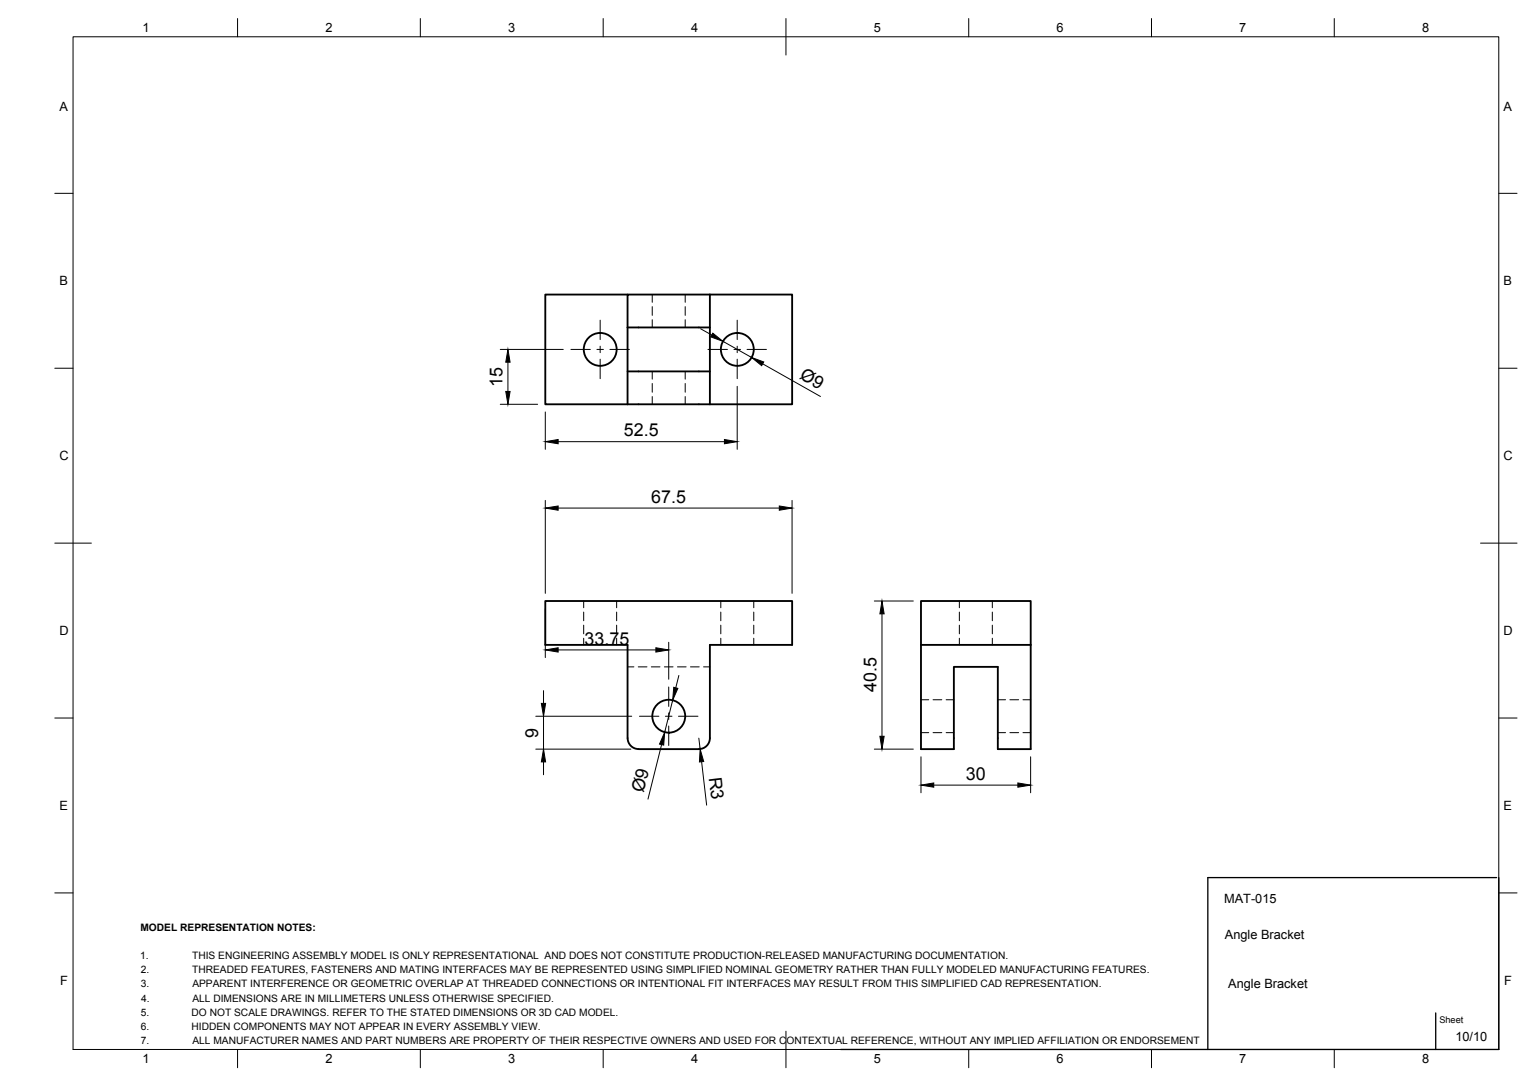
ISO-10303-21;
HEADER;
/* Generated by software containing ST-Developer
 * from STEP Tools, Inc. (www.steptools.com) 
 */

FILE_DESCRIPTION(
/* description */ ('STEP AP214'),
/* implementation_level */ '2;1');

FILE_NAME(
/* name */ 'Angle Bracket.step',
/* time_stamp */ '2026-11-14T06:03:18-08:00',
/* author */ (''),
/* organization */ (''),
/* preprocessor_version */ 'ST-DEVELOPER v20.2',
/* originating_system */ 'Autodesk Translation Framework v15.17.0.0',
/* authorisation */ '');

FILE_SCHEMA (('AUTOMOTIVE_DESIGN { 1 0 10303 214 3 1 1 }'));
ENDSEC;

DATA;
#10=MECHANICAL_DESIGN_GEOMETRIC_PRESENTATION_REPRESENTATION('',(#78),#3206);
#62=SHAPE_REPRESENTATION_RELATIONSHIP('SRR','None',#3245,#70);
#70=ADVANCED_BREP_SHAPE_REPRESENTATION('',(#86),#3204);
#78=STYLED_ITEM('',(#3290),#86);
#86=MANIFOLD_SOLID_BREP('Body1',#1785);
#131=PLANE('',#2029);
#132=PLANE('',#2030);
#133=PLANE('',#2031);
#134=PLANE('',#2032);
#135=PLANE('',#2033);
#136=PLANE('',#2034);
#137=PLANE('',#2037);
#138=PLANE('',#2038);
#139=PLANE('',#2041);
#140=PLANE('',#2042);
#141=PLANE('',#2043);
#142=PLANE('',#2044);
#143=PLANE('',#2047);
#144=PLANE('',#2050);
#180=FACE_BOUND('',#724,.T.);
#181=FACE_BOUND('',#726,.T.);
#182=FACE_BOUND('',#728,.T.);
#183=FACE_BOUND('',#729,.T.);
#184=FACE_BOUND('',#732,.T.);
#185=FACE_BOUND('',#735,.T.);
#186=FACE_BOUND('',#740,.T.);
#187=FACE_BOUND('',#742,.T.);
#286=LINE('',#3041,#431);
#287=LINE('',#3047,#432);
#288=LINE('',#3053,#433);
#289=LINE('',#3059,#434);
#290=LINE('',#3064,#435);
#291=LINE('',#3066,#436);
#292=LINE('',#3068,#437);
#293=LINE('',#3069,#438);
#294=LINE('',#3073,#439);
#295=LINE('',#3075,#440);
#296=LINE('',#3077,#441);
#297=LINE('',#3078,#442);
#298=LINE('',#3082,#443);
#299=LINE('',#3084,#444);
#300=LINE('',#3086,#445);
#301=LINE('',#3087,#446);
#302=LINE('',#3091,#447);
#303=LINE('',#3093,#448);
#304=LINE('',#3095,#449);
#305=LINE('',#3096,#450);
#306=LINE('',#3098,#451);
#307=LINE('',#3099,#452);
#308=LINE('',#3102,#453);
#309=LINE('',#3106,#454);
#310=LINE('',#3107,#455);
#311=LINE('',#3109,#456);
#312=LINE('',#3113,#457);
#313=LINE('',#3116,#458);
#314=LINE('',#3118,#459);
#315=LINE('',#3123,#460);
#316=LINE('',#3124,#461);
#317=LINE('',#3126,#462);
#318=LINE('',#3128,#463);
#319=LINE('',#3129,#464);
#320=LINE('',#3132,#465);
#321=LINE('',#3134,#466);
#322=LINE('',#3136,#467);
#323=LINE('',#3138,#468);
#324=LINE('',#3139,#469);
#325=LINE('',#3143,#470);
#326=LINE('',#3144,#471);
#327=LINE('',#3145,#472);
#328=LINE('',#3148,#473);
#329=LINE('',#3153,#474);
#431=VECTOR('',#2459,4.50000000000001);
#432=VECTOR('',#2466,4.50000000000001);
#433=VECTOR('',#2473,4.50000000000002);
#434=VECTOR('',#2480,4.50000000000001);
#435=VECTOR('',#2485,1000.);
#436=VECTOR('',#2486,1000.);
#437=VECTOR('',#2487,1000.);
#438=VECTOR('',#2488,1000.);
#439=VECTOR('',#2491,1000.);
#440=VECTOR('',#2492,1000.);
#441=VECTOR('',#2493,1000.);
#442=VECTOR('',#2494,1000.);
#443=VECTOR('',#2497,1000.);
#444=VECTOR('',#2498,1000.);
#445=VECTOR('',#2499,1000.);
#446=VECTOR('',#2500,1000.);
#447=VECTOR('',#2503,1000.);
#448=VECTOR('',#2504,1000.);
#449=VECTOR('',#2505,1000.);
#450=VECTOR('',#2506,1000.);
#451=VECTOR('',#2509,1000.);
#452=VECTOR('',#2510,1000.);
#453=VECTOR('',#2513,1000.);
#454=VECTOR('',#2518,1000.);
#455=VECTOR('',#2519,1000.);
#456=VECTOR('',#2522,1000.);
#457=VECTOR('',#2525,1000.);
#458=VECTOR('',#2528,1000.);
#459=VECTOR('',#2529,1000.);
#460=VECTOR('',#2534,1000.);
#461=VECTOR('',#2535,1000.);
#462=VECTOR('',#2536,1000.);
#463=VECTOR('',#2537,1000.);
#464=VECTOR('',#2538,1000.);
#465=VECTOR('',#2541,1000.);
#466=VECTOR('',#2542,1000.);
#467=VECTOR('',#2543,1000.);
#468=VECTOR('',#2544,1000.);
#469=VECTOR('',#2545,1000.);
#470=VECTOR('',#2548,1000.);
#471=VECTOR('',#2549,1000.);
#472=VECTOR('',#2550,1000.);
#473=VECTOR('',#2555,1000.);
#474=VECTOR('',#2564,1000.);
#503=CYLINDRICAL_SURFACE('',#2017,4.50000000000001);
#504=CYLINDRICAL_SURFACE('',#2020,4.50000000000001);
#505=CYLINDRICAL_SURFACE('',#2023,4.50000000000002);
#506=CYLINDRICAL_SURFACE('',#2026,4.50000000000001);
#507=CYLINDRICAL_SURFACE('',#2051,3.00000000000001);
#508=CYLINDRICAL_SURFACE('',#2052,3.00000000000001);
#509=CYLINDRICAL_SURFACE('',#2053,3.00000000000001);
#510=CYLINDRICAL_SURFACE('',#2054,3.00000000000001);
#585=FACE_OUTER_BOUND('',#718,.T.);
#586=FACE_OUTER_BOUND('',#719,.T.);
#587=FACE_OUTER_BOUND('',#720,.T.);
#588=FACE_OUTER_BOUND('',#721,.T.);
#589=FACE_OUTER_BOUND('',#722,.T.);
#590=FACE_OUTER_BOUND('',#723,.T.);
#591=FACE_OUTER_BOUND('',#725,.T.);
#592=FACE_OUTER_BOUND('',#727,.T.);
#593=FACE_OUTER_BOUND('',#730,.T.);
#594=FACE_OUTER_BOUND('',#731,.T.);
#595=FACE_OUTER_BOUND('',#733,.T.);
#596=FACE_OUTER_BOUND('',#734,.T.);
#597=FACE_OUTER_BOUND('',#736,.T.);
#598=FACE_OUTER_BOUND('',#737,.T.);
#599=FACE_OUTER_BOUND('',#738,.T.);
#600=FACE_OUTER_BOUND('',#739,.T.);
#601=FACE_OUTER_BOUND('',#741,.T.);
#602=FACE_OUTER_BOUND('',#743,.T.);
#603=FACE_OUTER_BOUND('',#744,.T.);
#604=FACE_OUTER_BOUND('',#745,.T.);
#605=FACE_OUTER_BOUND('',#746,.T.);
#606=FACE_OUTER_BOUND('',#747,.T.);
#718=EDGE_LOOP('',(#1541,#1542,#1543,#1544));
#719=EDGE_LOOP('',(#1545,#1546,#1547,#1548));
#720=EDGE_LOOP('',(#1549,#1550,#1551,#1552));
#721=EDGE_LOOP('',(#1553,#1554,#1555,#1556));
#722=EDGE_LOOP('',(#1557,#1558,#1559,#1560));
#723=EDGE_LOOP('',(#1561,#1562,#1563,#1564));
#724=EDGE_LOOP('',(#1565));
#725=EDGE_LOOP('',(#1566,#1567,#1568,#1569));
#726=EDGE_LOOP('',(#1570));
#727=EDGE_LOOP('',(#1571,#1572,#1573,#1574));
#728=EDGE_LOOP('',(#1575));
#729=EDGE_LOOP('',(#1576));
#730=EDGE_LOOP('',(#1577,#1578,#1579,#1580));
#731=EDGE_LOOP('',(#1581,#1582,#1583,#1584,#1585,#1586,#1587,#1588,#1589,
#1590));
#732=EDGE_LOOP('',(#1591));
#733=EDGE_LOOP('',(#1592,#1593,#1594,#1595));
#734=EDGE_LOOP('',(#1596,#1597,#1598,#1599,#1600,#1601,#1602,#1603,#1604,
#1605));
#735=EDGE_LOOP('',(#1606));
#736=EDGE_LOOP('',(#1607,#1608,#1609,#1610,#1611,#1612,#1613,#1614));
#737=EDGE_LOOP('',(#1615,#1616,#1617,#1618,#1619,#1620,#1621,#1622));
#738=EDGE_LOOP('',(#1623,#1624,#1625,#1626));
#739=EDGE_LOOP('',(#1627,#1628,#1629,#1630,#1631,#1632));
#740=EDGE_LOOP('',(#1633));
#741=EDGE_LOOP('',(#1634,#1635,#1636,#1637,#1638,#1639));
#742=EDGE_LOOP('',(#1640));
#743=EDGE_LOOP('',(#1641,#1642,#1643,#1644));
#744=EDGE_LOOP('',(#1645,#1646,#1647,#1648));
#745=EDGE_LOOP('',(#1649,#1650,#1651,#1652));
#746=EDGE_LOOP('',(#1653,#1654,#1655,#1656));
#747=EDGE_LOOP('',(#1657,#1658,#1659,#1660));
#813=CIRCLE('',#2018,4.50000000000001);
#814=CIRCLE('',#2019,4.50000000000001);
#815=CIRCLE('',#2021,4.50000000000001);
#816=CIRCLE('',#2022,4.50000000000001);
#817=CIRCLE('',#2024,4.50000000000002);
#818=CIRCLE('',#2025,4.50000000000002);
#819=CIRCLE('',#2027,4.50000000000001);
#820=CIRCLE('',#2028,4.50000000000001);
#821=CIRCLE('',#2035,3.00000000000001);
#822=CIRCLE('',#2036,3.00000000000001);
#823=CIRCLE('',#2039,3.00000000000001);
#824=CIRCLE('',#2040,3.00000000000001);
#825=CIRCLE('',#2045,3.00000000000001);
#826=CIRCLE('',#2046,3.00000000000001);
#827=CIRCLE('',#2048,3.00000000000001);
#828=CIRCLE('',#2049,3.00000000000001);
#942=VERTEX_POINT('',#3038);
#943=VERTEX_POINT('',#3040);
#944=VERTEX_POINT('',#3044);
#945=VERTEX_POINT('',#3046);
#946=VERTEX_POINT('',#3050);
#947=VERTEX_POINT('',#3052);
#948=VERTEX_POINT('',#3056);
#949=VERTEX_POINT('',#3058);
#950=VERTEX_POINT('',#3062);
#951=VERTEX_POINT('',#3063);
#952=VERTEX_POINT('',#3065);
#953=VERTEX_POINT('',#3067);
#954=VERTEX_POINT('',#3071);
#955=VERTEX_POINT('',#3072);
#956=VERTEX_POINT('',#3074);
#957=VERTEX_POINT('',#3076);
#958=VERTEX_POINT('',#3080);
#959=VERTEX_POINT('',#3081);
#960=VERTEX_POINT('',#3083);
#961=VERTEX_POINT('',#3085);
#962=VERTEX_POINT('',#3089);
#963=VERTEX_POINT('',#3090);
#964=VERTEX_POINT('',#3092);
#965=VERTEX_POINT('',#3094);
#966=VERTEX_POINT('',#3101);
#967=VERTEX_POINT('',#3104);
#968=VERTEX_POINT('',#3111);
#969=VERTEX_POINT('',#3112);
#970=VERTEX_POINT('',#3114);
#971=VERTEX_POINT('',#3117);
#972=VERTEX_POINT('',#3121);
#973=VERTEX_POINT('',#3122);
#974=VERTEX_POINT('',#3125);
#975=VERTEX_POINT('',#3127);
#976=VERTEX_POINT('',#3131);
#977=VERTEX_POINT('',#3133);
#978=VERTEX_POINT('',#3135);
#979=VERTEX_POINT('',#3137);
#980=VERTEX_POINT('',#3141);
#981=VERTEX_POINT('',#3142);
#1149=EDGE_CURVE('',#942,#942,#813,.T.);
#1150=EDGE_CURVE('',#942,#943,#286,.T.);
#1151=EDGE_CURVE('',#943,#943,#814,.T.);
#1152=EDGE_CURVE('',#944,#944,#815,.T.);
#1153=EDGE_CURVE('',#944,#945,#287,.T.);
#1154=EDGE_CURVE('',#945,#945,#816,.T.);
#1155=EDGE_CURVE('',#946,#946,#817,.T.);
#1156=EDGE_CURVE('',#946,#947,#288,.T.);
#1157=EDGE_CURVE('',#947,#947,#818,.T.);
#1158=EDGE_CURVE('',#948,#948,#819,.T.);
#1159=EDGE_CURVE('',#948,#949,#289,.T.);
#1160=EDGE_CURVE('',#949,#949,#820,.T.);
#1161=EDGE_CURVE('',#950,#951,#290,.T.);
#1162=EDGE_CURVE('',#951,#952,#291,.T.);
#1163=EDGE_CURVE('',#953,#952,#292,.T.);
#1164=EDGE_CURVE('',#953,#950,#293,.T.);
#1165=EDGE_CURVE('',#954,#955,#294,.T.);
#1166=EDGE_CURVE('',#954,#956,#295,.T.);
#1167=EDGE_CURVE('',#956,#957,#296,.T.);
#1168=EDGE_CURVE('',#957,#955,#297,.T.);
#1169=EDGE_CURVE('',#958,#959,#298,.T.);
#1170=EDGE_CURVE('',#958,#960,#299,.T.);
#1171=EDGE_CURVE('',#960,#961,#300,.T.);
#1172=EDGE_CURVE('',#961,#959,#301,.T.);
#1173=EDGE_CURVE('',#962,#963,#302,.T.);
#1174=EDGE_CURVE('',#964,#962,#303,.T.);
#1175=EDGE_CURVE('',#965,#964,#304,.T.);
#1176=EDGE_CURVE('',#963,#965,#305,.T.);
#1177=EDGE_CURVE('',#961,#963,#306,.T.);
#1178=EDGE_CURVE('',#960,#962,#307,.T.);
#1179=EDGE_CURVE('',#966,#954,#308,.T.);
#1180=EDGE_CURVE('',#966,#951,#821,.T.);
#1181=EDGE_CURVE('',#950,#967,#822,.T.);
#1182=EDGE_CURVE('',#967,#959,#309,.T.);
#1183=EDGE_CURVE('',#956,#965,#310,.T.);
#1184=EDGE_CURVE('',#957,#964,#311,.T.);
#1185=EDGE_CURVE('',#968,#969,#312,.T.);
#1186=EDGE_CURVE('',#968,#970,#823,.T.);
#1187=EDGE_CURVE('',#970,#955,#313,.T.);
#1188=EDGE_CURVE('',#971,#958,#314,.T.);
#1189=EDGE_CURVE('',#971,#969,#824,.T.);
#1190=EDGE_CURVE('',#972,#973,#315,.T.);
#1191=EDGE_CURVE('',#973,#971,#316,.T.);
#1192=EDGE_CURVE('',#967,#974,#317,.T.);
#1193=EDGE_CURVE('',#975,#974,#318,.T.);
#1194=EDGE_CURVE('',#972,#975,#319,.T.);
#1195=EDGE_CURVE('',#970,#976,#320,.T.);
#1196=EDGE_CURVE('',#977,#976,#321,.T.);
#1197=EDGE_CURVE('',#978,#977,#322,.T.);
#1198=EDGE_CURVE('',#978,#979,#323,.T.);
#1199=EDGE_CURVE('',#979,#966,#324,.T.);
#1200=EDGE_CURVE('',#980,#981,#325,.T.);
#1201=EDGE_CURVE('',#980,#968,#326,.T.);
#1202=EDGE_CURVE('',#969,#981,#327,.T.);
#1203=EDGE_CURVE('',#952,#979,#825,.T.);
#1204=EDGE_CURVE('',#975,#978,#328,.T.);
#1205=EDGE_CURVE('',#974,#953,#826,.T.);
#1206=EDGE_CURVE('',#976,#980,#827,.T.);
#1207=EDGE_CURVE('',#981,#973,#828,.T.);
#1208=EDGE_CURVE('',#977,#972,#329,.T.);
#1541=ORIENTED_EDGE('',*,*,#1149,.F.);
#1542=ORIENTED_EDGE('',*,*,#1150,.T.);
#1543=ORIENTED_EDGE('',*,*,#1151,.T.);
#1544=ORIENTED_EDGE('',*,*,#1150,.F.);
#1545=ORIENTED_EDGE('',*,*,#1152,.F.);
#1546=ORIENTED_EDGE('',*,*,#1153,.T.);
#1547=ORIENTED_EDGE('',*,*,#1154,.F.);
#1548=ORIENTED_EDGE('',*,*,#1153,.F.);
#1549=ORIENTED_EDGE('',*,*,#1155,.T.);
#1550=ORIENTED_EDGE('',*,*,#1156,.T.);
#1551=ORIENTED_EDGE('',*,*,#1157,.F.);
#1552=ORIENTED_EDGE('',*,*,#1156,.F.);
#1553=ORIENTED_EDGE('',*,*,#1158,.T.);
#1554=ORIENTED_EDGE('',*,*,#1159,.T.);
#1555=ORIENTED_EDGE('',*,*,#1160,.F.);
#1556=ORIENTED_EDGE('',*,*,#1159,.F.);
#1557=ORIENTED_EDGE('',*,*,#1161,.T.);
#1558=ORIENTED_EDGE('',*,*,#1162,.T.);
#1559=ORIENTED_EDGE('',*,*,#1163,.F.);
#1560=ORIENTED_EDGE('',*,*,#1164,.T.);
#1561=ORIENTED_EDGE('',*,*,#1165,.F.);
#1562=ORIENTED_EDGE('',*,*,#1166,.T.);
#1563=ORIENTED_EDGE('',*,*,#1167,.T.);
#1564=ORIENTED_EDGE('',*,*,#1168,.T.);
#1565=ORIENTED_EDGE('',*,*,#1155,.F.);
#1566=ORIENTED_EDGE('',*,*,#1169,.F.);
#1567=ORIENTED_EDGE('',*,*,#1170,.T.);
#1568=ORIENTED_EDGE('',*,*,#1171,.T.);
#1569=ORIENTED_EDGE('',*,*,#1172,.T.);
#1570=ORIENTED_EDGE('',*,*,#1158,.F.);
#1571=ORIENTED_EDGE('',*,*,#1173,.F.);
#1572=ORIENTED_EDGE('',*,*,#1174,.F.);
#1573=ORIENTED_EDGE('',*,*,#1175,.F.);
#1574=ORIENTED_EDGE('',*,*,#1176,.F.);
#1575=ORIENTED_EDGE('',*,*,#1157,.T.);
#1576=ORIENTED_EDGE('',*,*,#1160,.T.);
#1577=ORIENTED_EDGE('',*,*,#1173,.T.);
#1578=ORIENTED_EDGE('',*,*,#1177,.F.);
#1579=ORIENTED_EDGE('',*,*,#1171,.F.);
#1580=ORIENTED_EDGE('',*,*,#1178,.T.);
#1581=ORIENTED_EDGE('',*,*,#1179,.F.);
#1582=ORIENTED_EDGE('',*,*,#1180,.T.);
#1583=ORIENTED_EDGE('',*,*,#1161,.F.);
#1584=ORIENTED_EDGE('',*,*,#1181,.T.);
#1585=ORIENTED_EDGE('',*,*,#1182,.T.);
#1586=ORIENTED_EDGE('',*,*,#1172,.F.);
#1587=ORIENTED_EDGE('',*,*,#1177,.T.);
#1588=ORIENTED_EDGE('',*,*,#1176,.T.);
#1589=ORIENTED_EDGE('',*,*,#1183,.F.);
#1590=ORIENTED_EDGE('',*,*,#1166,.F.);
#1591=ORIENTED_EDGE('',*,*,#1151,.F.);
#1592=ORIENTED_EDGE('',*,*,#1175,.T.);
#1593=ORIENTED_EDGE('',*,*,#1184,.F.);
#1594=ORIENTED_EDGE('',*,*,#1167,.F.);
#1595=ORIENTED_EDGE('',*,*,#1183,.T.);
#1596=ORIENTED_EDGE('',*,*,#1185,.F.);
#1597=ORIENTED_EDGE('',*,*,#1186,.T.);
#1598=ORIENTED_EDGE('',*,*,#1187,.T.);
#1599=ORIENTED_EDGE('',*,*,#1168,.F.);
#1600=ORIENTED_EDGE('',*,*,#1184,.T.);
#1601=ORIENTED_EDGE('',*,*,#1174,.T.);
#1602=ORIENTED_EDGE('',*,*,#1178,.F.);
#1603=ORIENTED_EDGE('',*,*,#1170,.F.);
#1604=ORIENTED_EDGE('',*,*,#1188,.F.);
#1605=ORIENTED_EDGE('',*,*,#1189,.T.);
#1606=ORIENTED_EDGE('',*,*,#1152,.T.);
#1607=ORIENTED_EDGE('',*,*,#1190,.T.);
#1608=ORIENTED_EDGE('',*,*,#1191,.T.);
#1609=ORIENTED_EDGE('',*,*,#1188,.T.);
#1610=ORIENTED_EDGE('',*,*,#1169,.T.);
#1611=ORIENTED_EDGE('',*,*,#1182,.F.);
#1612=ORIENTED_EDGE('',*,*,#1192,.T.);
#1613=ORIENTED_EDGE('',*,*,#1193,.F.);
#1614=ORIENTED_EDGE('',*,*,#1194,.F.);
#1615=ORIENTED_EDGE('',*,*,#1187,.F.);
#1616=ORIENTED_EDGE('',*,*,#1195,.T.);
#1617=ORIENTED_EDGE('',*,*,#1196,.F.);
#1618=ORIENTED_EDGE('',*,*,#1197,.F.);
#1619=ORIENTED_EDGE('',*,*,#1198,.T.);
#1620=ORIENTED_EDGE('',*,*,#1199,.T.);
#1621=ORIENTED_EDGE('',*,*,#1179,.T.);
#1622=ORIENTED_EDGE('',*,*,#1165,.T.);
#1623=ORIENTED_EDGE('',*,*,#1200,.F.);
#1624=ORIENTED_EDGE('',*,*,#1201,.T.);
#1625=ORIENTED_EDGE('',*,*,#1185,.T.);
#1626=ORIENTED_EDGE('',*,*,#1202,.T.);
#1627=ORIENTED_EDGE('',*,*,#1163,.T.);
#1628=ORIENTED_EDGE('',*,*,#1203,.T.);
#1629=ORIENTED_EDGE('',*,*,#1198,.F.);
#1630=ORIENTED_EDGE('',*,*,#1204,.F.);
#1631=ORIENTED_EDGE('',*,*,#1193,.T.);
#1632=ORIENTED_EDGE('',*,*,#1205,.T.);
#1633=ORIENTED_EDGE('',*,*,#1149,.T.);
#1634=ORIENTED_EDGE('',*,*,#1196,.T.);
#1635=ORIENTED_EDGE('',*,*,#1206,.T.);
#1636=ORIENTED_EDGE('',*,*,#1200,.T.);
#1637=ORIENTED_EDGE('',*,*,#1207,.T.);
#1638=ORIENTED_EDGE('',*,*,#1190,.F.);
#1639=ORIENTED_EDGE('',*,*,#1208,.F.);
#1640=ORIENTED_EDGE('',*,*,#1154,.T.);
#1641=ORIENTED_EDGE('',*,*,#1197,.T.);
#1642=ORIENTED_EDGE('',*,*,#1208,.T.);
#1643=ORIENTED_EDGE('',*,*,#1194,.T.);
#1644=ORIENTED_EDGE('',*,*,#1204,.T.);
#1645=ORIENTED_EDGE('',*,*,#1206,.F.);
#1646=ORIENTED_EDGE('',*,*,#1195,.F.);
#1647=ORIENTED_EDGE('',*,*,#1186,.F.);
#1648=ORIENTED_EDGE('',*,*,#1201,.F.);
#1649=ORIENTED_EDGE('',*,*,#1180,.F.);
#1650=ORIENTED_EDGE('',*,*,#1199,.F.);
#1651=ORIENTED_EDGE('',*,*,#1203,.F.);
#1652=ORIENTED_EDGE('',*,*,#1162,.F.);
#1653=ORIENTED_EDGE('',*,*,#1189,.F.);
#1654=ORIENTED_EDGE('',*,*,#1191,.F.);
#1655=ORIENTED_EDGE('',*,*,#1207,.F.);
#1656=ORIENTED_EDGE('',*,*,#1202,.F.);
#1657=ORIENTED_EDGE('',*,*,#1205,.F.);
#1658=ORIENTED_EDGE('',*,*,#1192,.F.);
#1659=ORIENTED_EDGE('',*,*,#1181,.F.);
#1660=ORIENTED_EDGE('',*,*,#1164,.F.);
#1752=ADVANCED_FACE('',(#585),#503,.F.);
#1753=ADVANCED_FACE('',(#586),#504,.F.);
#1754=ADVANCED_FACE('',(#587),#505,.F.);
#1755=ADVANCED_FACE('',(#588),#506,.F.);
#1756=ADVANCED_FACE('',(#589),#131,.F.);
#1757=ADVANCED_FACE('',(#590,#180),#132,.T.);
#1758=ADVANCED_FACE('',(#591,#181),#133,.T.);
#1759=ADVANCED_FACE('',(#592,#182,#183),#134,.F.);
#1760=ADVANCED_FACE('',(#593),#135,.F.);
#1761=ADVANCED_FACE('',(#594,#184),#136,.F.);
#1762=ADVANCED_FACE('',(#595),#137,.F.);
#1763=ADVANCED_FACE('',(#596,#185),#138,.F.);
#1764=ADVANCED_FACE('',(#597),#139,.F.);
#1765=ADVANCED_FACE('',(#598),#140,.F.);
#1766=ADVANCED_FACE('',(#599),#141,.F.);
#1767=ADVANCED_FACE('',(#600,#186),#142,.F.);
#1768=ADVANCED_FACE('',(#601,#187),#143,.F.);
#1769=ADVANCED_FACE('',(#602),#144,.T.);
#1770=ADVANCED_FACE('',(#603),#507,.T.);
#1771=ADVANCED_FACE('',(#604),#508,.T.);
#1772=ADVANCED_FACE('',(#605),#509,.T.);
#1773=ADVANCED_FACE('',(#606),#510,.T.);
#1785=CLOSED_SHELL('',(#1752,#1753,#1754,#1755,#1756,#1757,#1758,#1759,
#1760,#1761,#1762,#1763,#1764,#1765,#1766,#1767,#1768,#1769,#1770,#1771,
#1772,#1773));
#2016=AXIS2_PLACEMENT_3D('',#3036,#2453,#2454);
#2017=AXIS2_PLACEMENT_3D('',#3037,#2455,#2456);
#2018=AXIS2_PLACEMENT_3D('',#3039,#2457,#2458);
#2019=AXIS2_PLACEMENT_3D('',#3042,#2460,#2461);
#2020=AXIS2_PLACEMENT_3D('',#3043,#2462,#2463);
#2021=AXIS2_PLACEMENT_3D('',#3045,#2464,#2465);
#2022=AXIS2_PLACEMENT_3D('',#3048,#2467,#2468);
#2023=AXIS2_PLACEMENT_3D('',#3049,#2469,#2470);
#2024=AXIS2_PLACEMENT_3D('',#3051,#2471,#2472);
#2025=AXIS2_PLACEMENT_3D('',#3054,#2474,#2475);
#2026=AXIS2_PLACEMENT_3D('',#3055,#2476,#2477);
#2027=AXIS2_PLACEMENT_3D('',#3057,#2478,#2479);
#2028=AXIS2_PLACEMENT_3D('',#3060,#2481,#2482);
#2029=AXIS2_PLACEMENT_3D('',#3061,#2483,#2484);
#2030=AXIS2_PLACEMENT_3D('',#3070,#2489,#2490);
#2031=AXIS2_PLACEMENT_3D('',#3079,#2495,#2496);
#2032=AXIS2_PLACEMENT_3D('',#3088,#2501,#2502);
#2033=AXIS2_PLACEMENT_3D('',#3097,#2507,#2508);
#2034=AXIS2_PLACEMENT_3D('',#3100,#2511,#2512);
#2035=AXIS2_PLACEMENT_3D('',#3103,#2514,#2515);
#2036=AXIS2_PLACEMENT_3D('',#3105,#2516,#2517);
#2037=AXIS2_PLACEMENT_3D('',#3108,#2520,#2521);
#2038=AXIS2_PLACEMENT_3D('',#3110,#2523,#2524);
#2039=AXIS2_PLACEMENT_3D('',#3115,#2526,#2527);
#2040=AXIS2_PLACEMENT_3D('',#3119,#2530,#2531);
#2041=AXIS2_PLACEMENT_3D('',#3120,#2532,#2533);
#2042=AXIS2_PLACEMENT_3D('',#3130,#2539,#2540);
#2043=AXIS2_PLACEMENT_3D('',#3140,#2546,#2547);
#2044=AXIS2_PLACEMENT_3D('',#3146,#2551,#2552);
#2045=AXIS2_PLACEMENT_3D('',#3147,#2553,#2554);
#2046=AXIS2_PLACEMENT_3D('',#3149,#2556,#2557);
#2047=AXIS2_PLACEMENT_3D('',#3150,#2558,#2559);
#2048=AXIS2_PLACEMENT_3D('',#3151,#2560,#2561);
#2049=AXIS2_PLACEMENT_3D('',#3152,#2562,#2563);
#2050=AXIS2_PLACEMENT_3D('',#3154,#2565,#2566);
#2051=AXIS2_PLACEMENT_3D('',#3155,#2567,#2568);
#2052=AXIS2_PLACEMENT_3D('',#3156,#2569,#2570);
#2053=AXIS2_PLACEMENT_3D('',#3157,#2571,#2572);
#2054=AXIS2_PLACEMENT_3D('',#3158,#2573,#2574);
#2453=DIRECTION('axis',(0.,0.,1.));
#2454=DIRECTION('refdir',(1.,0.,0.));
#2455=DIRECTION('center_axis',(-2.9274135154686E-32,-1.,1.84552236920907E-31));
#2456=DIRECTION('ref_axis',(-5.40260712672226E-63,-1.84552236920907E-31,
-1.));
#2457=DIRECTION('center_axis',(-2.9274135154686E-32,-1.,1.84552236920907E-31));
#2458=DIRECTION('ref_axis',(-5.40260712672226E-63,-1.84552236920907E-31,
-1.));
#2459=DIRECTION('',(-2.9274135154686E-32,-1.,1.84552236920907E-31));
#2460=DIRECTION('center_axis',(-2.9274135154686E-32,-1.,1.84552236920907E-31));
#2461=DIRECTION('ref_axis',(-5.40260712672226E-63,-1.84552236920907E-31,
-1.));
#2462=DIRECTION('center_axis',(-2.9274135154686E-32,-1.,1.84552236920907E-31));
#2463=DIRECTION('ref_axis',(-5.40260712672226E-63,-1.84552236920907E-31,
-1.));
#2464=DIRECTION('center_axis',(-2.9274135154686E-32,-1.,1.84552236920907E-31));
#2465=DIRECTION('ref_axis',(-5.40260712672226E-63,-1.84552236920907E-31,
-1.));
#2466=DIRECTION('',(-2.9274135154686E-32,-1.,1.84552236920907E-31));
#2467=DIRECTION('center_axis',(2.9274135154686E-32,1.,-1.84552236920907E-31));
#2468=DIRECTION('ref_axis',(5.40260712672226E-63,1.84552236920907E-31,1.));
#2469=DIRECTION('center_axis',(1.04083408558608E-17,1.72178137028218E-31,
-1.));
#2470=DIRECTION('ref_axis',(-1.,1.79208873811681E-48,-1.04083408558608E-17));
#2471=DIRECTION('center_axis',(-1.04083408558608E-17,-1.72178137028218E-31,
1.));
#2472=DIRECTION('ref_axis',(-1.,1.79208873811681E-48,-1.04083408558608E-17));
#2473=DIRECTION('',(1.04083408558608E-17,1.72178137028218E-31,-1.));
#2474=DIRECTION('center_axis',(-1.04083408558608E-17,-1.72178137028218E-31,
1.));
#2475=DIRECTION('ref_axis',(-1.,1.79208873811681E-48,-1.04083408558608E-17));
#2476=DIRECTION('center_axis',(1.04083408558608E-17,1.72178137028218E-31,
-1.));
#2477=DIRECTION('ref_axis',(-1.,1.79208873811681E-48,-1.04083408558608E-17));
#2478=DIRECTION('center_axis',(-1.04083408558608E-17,-1.72178137028218E-31,
1.));
#2479=DIRECTION('ref_axis',(1.,-1.79208873811681E-48,1.04083408558608E-17));
#2480=DIRECTION('',(1.04083408558608E-17,1.72178137028218E-31,-1.));
#2481=DIRECTION('center_axis',(-1.04083408558608E-17,-1.72178137028218E-31,
1.));
#2482=DIRECTION('ref_axis',(1.,-1.79208873811681E-48,1.04083408558608E-17));
#2483=DIRECTION('center_axis',(1.04083408558608E-17,1.72178137028218E-31,
-1.));
#2484=DIRECTION('ref_axis',(-1.,-2.77333911991761E-32,-1.04083408558608E-17));
#2485=DIRECTION('',(1.,2.77333911991761E-32,1.04083408558608E-17));
#2486=DIRECTION('',(2.9274135154686E-32,1.,-1.84552236920907E-31));
#2487=DIRECTION('',(1.,2.77333911991761E-32,1.04083408558608E-17));
#2488=DIRECTION('',(-2.9274135154686E-32,-1.,1.84552236920907E-31));
#2489=DIRECTION('center_axis',(-1.04083408558608E-17,-1.72178137028218E-31,
1.));
#2490=DIRECTION('ref_axis',(1.,2.77333911991761E-32,1.04083408558608E-17));
#2491=DIRECTION('',(2.9274135154686E-32,1.,-1.84552236920907E-31));
#2492=DIRECTION('',(1.,2.92741351546859E-32,6.93889390390721E-18));
#2493=DIRECTION('',(2.9274135154686E-32,1.,-1.84552236920907E-31));
#2494=DIRECTION('',(-1.,-2.77333911991761E-32,-1.04083408558608E-17));
#2495=DIRECTION('center_axis',(-1.04083408558608E-17,-1.72178137028218E-31,
1.));
#2496=DIRECTION('ref_axis',(1.,2.77333911991761E-32,1.04083408558608E-17));
#2497=DIRECTION('',(-2.9274135154686E-32,-1.,1.84552236920907E-31));
#2498=DIRECTION('',(-1.,-2.77333911991761E-32,-1.04083408558608E-17));
#2499=DIRECTION('',(-2.9274135154686E-32,-1.,1.84552236920907E-31));
#2500=DIRECTION('',(1.,2.92741351546859E-32,6.93889390390721E-18));
#2501=DIRECTION('center_axis',(-1.04083408558608E-17,-1.72178137028218E-31,
1.));
#2502=DIRECTION('ref_axis',(1.,2.77333911991761E-32,1.04083408558608E-17));
#2503=DIRECTION('',(-2.9274135154686E-32,-1.,1.84552236920907E-31));
#2504=DIRECTION('',(-1.,3.46944695195361E-16,-1.04083408558608E-17));
#2505=DIRECTION('',(2.9274135154686E-32,1.,-1.84552236920907E-31));
#2506=DIRECTION('',(1.,2.92741351546859E-32,6.93889390390721E-18));
#2507=DIRECTION('center_axis',(1.,2.77333911991761E-32,1.04083408558608E-17));
#2508=DIRECTION('ref_axis',(1.04083408558608E-17,1.72178137028218E-31,-1.));
#2509=DIRECTION('',(1.04083408558608E-17,1.72178137028218E-31,-1.));
#2510=DIRECTION('',(1.04083408558608E-17,1.72178137028218E-31,-1.));
#2511=DIRECTION('center_axis',(2.9274135154686E-32,1.,1.72178137028218E-31));
#2512=DIRECTION('ref_axis',(-1.04083408558608E-17,-1.72178137028218E-31,
1.));
#2513=DIRECTION('',(1.04083408558608E-17,1.72178137028218E-31,-1.));
#2514=DIRECTION('center_axis',(-2.9274135154686E-32,-1.,1.84552236920907E-31));
#2515=DIRECTION('ref_axis',(-4.85722573273504E-14,1.84552236920908E-31,
1.));
#2516=DIRECTION('center_axis',(-2.9274135154686E-32,-1.,1.84552236920907E-31));
#2517=DIRECTION('ref_axis',(5.40260712672226E-63,1.84552236920907E-31,1.));
#2518=DIRECTION('',(1.04083408558608E-17,1.72178137028218E-31,-1.));
#2519=DIRECTION('',(1.04083408558608E-17,1.72178137028218E-31,-1.));
#2520=DIRECTION('center_axis',(-1.,-2.77333911991761E-32,-1.04083408558608E-17));
#2521=DIRECTION('ref_axis',(-1.04083408558608E-17,-1.72178137028218E-31,
1.));
#2522=DIRECTION('',(1.04083408558608E-17,1.72178137028218E-31,-1.));
#2523=DIRECTION('center_axis',(-3.46944695195361E-16,-1.,1.4637067577343E-31));
#2524=DIRECTION('ref_axis',(1.,-3.46944695195361E-16,1.04083408558608E-17));
#2525=DIRECTION('',(-1.,-2.77333911991761E-32,-1.04083408558608E-17));
#2526=DIRECTION('center_axis',(3.46944695195362E-16,1.,-1.4637067577343E-31));
#2527=DIRECTION('ref_axis',(1.,-3.46944695195362E-16,3.4694469519536E-14));
#2528=DIRECTION('',(1.04083408558608E-17,1.72178137028218E-31,-1.));
#2529=DIRECTION('',(1.04083408558608E-17,1.72178137028218E-31,-1.));
#2530=DIRECTION('center_axis',(3.46944695195362E-16,1.,-1.4637067577343E-31));
#2531=DIRECTION('ref_axis',(1.,-3.46944695195362E-16,5.07825294917518E-47));
#2532=DIRECTION('center_axis',(1.,2.77333911991761E-32,1.04083408558608E-17));
#2533=DIRECTION('ref_axis',(1.04083408558608E-17,1.72178137028218E-31,-1.));
#2534=DIRECTION('',(-1.04083408558608E-17,-1.72178137028218E-31,1.));
#2535=DIRECTION('',(2.9274135154686E-32,1.,-1.84552236920907E-31));
#2536=DIRECTION('',(2.9274135154686E-32,1.,-1.84552236920907E-31));
#2537=DIRECTION('',(-1.04083408558608E-17,-1.72178137028218E-31,1.));
#2538=DIRECTION('',(-2.9274135154686E-32,-1.,1.84552236920907E-31));
#2539=DIRECTION('center_axis',(-1.,-2.77333911991761E-32,-1.04083408558608E-17));
#2540=DIRECTION('ref_axis',(-1.04083408558608E-17,-1.72178137028218E-31,
1.));
#2541=DIRECTION('',(-2.9274135154686E-32,-1.,1.84552236920907E-31));
#2542=DIRECTION('',(-1.04083408558608E-17,-1.72178137028218E-31,1.));
#2543=DIRECTION('',(2.9274135154686E-32,1.,-1.84552236920907E-31));
#2544=DIRECTION('',(-1.04083408558608E-17,-1.72178137028218E-31,1.));
#2545=DIRECTION('',(-2.9274135154686E-32,-1.,1.84552236920907E-31));
#2546=DIRECTION('center_axis',(1.04083408558608E-17,1.72178137028218E-31,
-1.));
#2547=DIRECTION('ref_axis',(-1.,-2.77333911991761E-32,-1.04083408558608E-17));
#2548=DIRECTION('',(-1.,-2.77333911991761E-32,-1.04083408558608E-17));
#2549=DIRECTION('',(2.9274135154686E-32,1.,-1.84552236920907E-31));
#2550=DIRECTION('',(-2.9274135154686E-32,-1.,1.84552236920907E-31));
#2551=DIRECTION('center_axis',(-2.9274135154686E-32,-1.,-1.72178137028218E-31));
#2552=DIRECTION('ref_axis',(1.04083408558608E-17,1.72178137028218E-31,-1.));
#2553=DIRECTION('center_axis',(2.9274135154686E-32,1.,-1.84552236920907E-31));
#2554=DIRECTION('ref_axis',(-5.40260712672226E-63,-1.84552236920907E-31,
-1.));
#2555=DIRECTION('',(1.,2.77333911991761E-32,1.04083408558608E-17));
#2556=DIRECTION('center_axis',(2.9274135154686E-32,1.,-1.84552236920907E-31));
#2557=DIRECTION('ref_axis',(-1.15648231731787E-15,-1.84552236920907E-31,
-1.));
#2558=DIRECTION('center_axis',(2.9274135154686E-32,1.,1.72178137028218E-31));
#2559=DIRECTION('ref_axis',(-1.04083408558608E-17,-1.72178137028218E-31,
1.));
#2560=DIRECTION('center_axis',(-2.9274135154686E-32,-1.,1.84552236920907E-31));
#2561=DIRECTION('ref_axis',(-4.85722573273504E-14,1.84552236920908E-31,
1.));
#2562=DIRECTION('center_axis',(-2.9274135154686E-32,-1.,1.84552236920907E-31));
#2563=DIRECTION('ref_axis',(5.40260712672226E-63,1.84552236920907E-31,1.));
#2564=DIRECTION('',(-1.,-2.77333911991761E-32,-1.04083408558608E-17));
#2565=DIRECTION('center_axis',(-1.04083408558608E-17,-1.72178137028218E-31,
1.));
#2566=DIRECTION('ref_axis',(1.,2.77333911991761E-32,1.04083408558608E-17));
#2567=DIRECTION('center_axis',(2.9274135154686E-32,1.,-1.84552236920907E-31));
#2568=DIRECTION('ref_axis',(5.40260712672226E-63,1.84552236920907E-31,1.));
#2569=DIRECTION('center_axis',(2.9274135154686E-32,1.,-1.84552236920907E-31));
#2570=DIRECTION('ref_axis',(5.40260712672226E-63,1.84552236920907E-31,1.));
#2571=DIRECTION('center_axis',(-2.9274135154686E-32,-1.,1.84552236920907E-31));
#2572=DIRECTION('ref_axis',(-5.40260712672226E-63,-1.84552236920907E-31,
-1.));
#2573=DIRECTION('center_axis',(-2.9274135154686E-32,-1.,1.84552236920907E-31));
#2574=DIRECTION('ref_axis',(-5.40260712672226E-63,-1.84552236920907E-31,
-1.));
#3036=CARTESIAN_POINT('',(0.,0.,0.));
#3037=CARTESIAN_POINT('Origin',(22.5,25.,27.4190038418755));
#3038=CARTESIAN_POINT('',(22.5,3.99999999999999,31.9190038418755));
#3039=CARTESIAN_POINT('Origin',(22.5,3.99999999999999,27.4190038418755));
#3040=CARTESIAN_POINT('',(22.5,-5.,31.9190038418755));
#3041=CARTESIAN_POINT('',(22.5,25.,31.9190038418755));
#3042=CARTESIAN_POINT('Origin',(22.5,-5.,27.4190038418755));
#3043=CARTESIAN_POINT('Origin',(22.5,25.,27.4190038418755));
#3044=CARTESIAN_POINT('',(22.5,25.,31.9190038418755));
#3045=CARTESIAN_POINT('Origin',(22.5,25.,27.4190038418755));
#3046=CARTESIAN_POINT('',(22.5,16.,31.9190038418755));
#3047=CARTESIAN_POINT('',(22.5,25.,31.9190038418755));
#3048=CARTESIAN_POINT('Origin',(22.5,16.,27.4190038418755));
#3049=CARTESIAN_POINT('Origin',(41.25,10.,7.91900384187549));
#3050=CARTESIAN_POINT('',(45.75,10.,7.91900384187549));
#3051=CARTESIAN_POINT('Origin',(41.25,10.,7.91900384187549));
#3052=CARTESIAN_POINT('',(45.75,10.,-4.0809961581245));
#3053=CARTESIAN_POINT('',(45.75,10.,7.91900384187549));
#3054=CARTESIAN_POINT('Origin',(41.25,10.,-4.0809961581245));
#3055=CARTESIAN_POINT('Origin',(3.74999999999999,10.,7.91900384187547));
#3056=CARTESIAN_POINT('',(8.25,10.,7.91900384187547));
#3057=CARTESIAN_POINT('Origin',(3.74999999999999,10.,7.91900384187547));
#3058=CARTESIAN_POINT('',(8.25,10.,-4.08099615812454));
#3059=CARTESIAN_POINT('',(8.25,10.,7.91900384187547));
#3060=CARTESIAN_POINT('Origin',(3.74999999999999,10.,-4.08099615812454));
#3061=CARTESIAN_POINT('Origin',(-11.25,-5.,36.4190038418755));
#3062=CARTESIAN_POINT('',(14.25,-5.,36.4190038418755));
#3063=CARTESIAN_POINT('',(30.7500000000001,-5.,36.4190038418755));
#3064=CARTESIAN_POINT('',(33.75,-5.,36.4190038418755));
#3065=CARTESIAN_POINT('',(30.7500000000001,3.99999999999999,36.4190038418755));
#3066=CARTESIAN_POINT('',(30.7500000000001,-5.,36.4190038418755));
#3067=CARTESIAN_POINT('',(14.25,3.99999999999999,36.4190038418755));
#3068=CARTESIAN_POINT('',(-11.25,3.99999999999999,36.4190038418755));
#3069=CARTESIAN_POINT('',(14.25,-5.,36.4190038418755));
#3070=CARTESIAN_POINT('Origin',(-11.2500000000001,-5.,7.91900384187547));
#3071=CARTESIAN_POINT('',(33.75,-5.,7.91900384187549));
#3072=CARTESIAN_POINT('',(33.75,25.,7.91900384187549));
#3073=CARTESIAN_POINT('',(33.75,25.,7.91900384187549));
#3074=CARTESIAN_POINT('',(56.2500000000001,-5.,7.91900384187549));
#3075=CARTESIAN_POINT('',(-11.2500000000001,-5.,7.91900384187547));
#3076=CARTESIAN_POINT('',(56.2500000000001,25.,7.91900384187549));
#3077=CARTESIAN_POINT('',(56.2500000000001,-5.,7.91900384187549));
#3078=CARTESIAN_POINT('',(56.2500000000001,25.,7.91900384187549));
#3079=CARTESIAN_POINT('Origin',(-11.2500000000001,-5.,7.91900384187547));
#3080=CARTESIAN_POINT('',(11.25,25.,7.91900384187549));
#3081=CARTESIAN_POINT('',(11.25,-5.,7.91900384187549));
#3082=CARTESIAN_POINT('',(11.25,25.,7.91900384187549));
#3083=CARTESIAN_POINT('',(-11.2500000000001,25.,7.91900384187547));
#3084=CARTESIAN_POINT('',(56.2500000000001,25.,7.91900384187549));
#3085=CARTESIAN_POINT('',(-11.2500000000001,-5.,7.91900384187547));
#3086=CARTESIAN_POINT('',(-11.2500000000001,25.,7.91900384187547));
#3087=CARTESIAN_POINT('',(-11.2500000000001,-5.,7.91900384187547));
#3088=CARTESIAN_POINT('Origin',(-11.25,-5.,-4.08099615812456));
#3089=CARTESIAN_POINT('',(-11.25,25.,-4.08099615812456));
#3090=CARTESIAN_POINT('',(-11.25,-5.,-4.08099615812456));
#3091=CARTESIAN_POINT('',(-11.25,25.,-4.08099615812456));
#3092=CARTESIAN_POINT('',(56.2500000000001,25.,-4.08099615812452));
#3093=CARTESIAN_POINT('',(3.74999999999999,25.,-4.08099615812456));
#3094=CARTESIAN_POINT('',(56.2500000000001,-5.,-4.0809961581245));
#3095=CARTESIAN_POINT('',(56.2500000000001,-5.,-4.0809961581245));
#3096=CARTESIAN_POINT('',(-11.25,-5.,-4.08099615812456));
#3097=CARTESIAN_POINT('Origin',(-11.2500000000001,25.,7.91900384187547));
#3098=CARTESIAN_POINT('',(-11.2500000000001,-5.,7.91900384187547));
#3099=CARTESIAN_POINT('',(-11.2500000000001,25.,7.91900384187547));
#3100=CARTESIAN_POINT('Origin',(-11.2500000000001,-5.,7.91900384187547));
#3101=CARTESIAN_POINT('',(33.75,-5.,33.4190038418755));
#3102=CARTESIAN_POINT('',(33.75,-5.,36.4190038418755));
#3103=CARTESIAN_POINT('Origin',(30.75,-5.,33.4190038418756));
#3104=CARTESIAN_POINT('',(11.25,-5.,33.4190038418756));
#3105=CARTESIAN_POINT('Origin',(14.25,-5.,33.4190038418756));
#3106=CARTESIAN_POINT('',(11.25,-5.,36.4190038418755));
#3107=CARTESIAN_POINT('',(56.2500000000001,-5.,7.91900384187549));
#3108=CARTESIAN_POINT('Origin',(56.2500000000001,-5.,7.91900384187549));
#3109=CARTESIAN_POINT('',(56.2500000000001,25.,7.91900384187549));
#3110=CARTESIAN_POINT('Origin',(3.74999999999999,25.,7.91900384187547));
#3111=CARTESIAN_POINT('',(30.7500000000001,25.,36.4190038418755));
#3112=CARTESIAN_POINT('',(14.25,25.,36.4190038418755));
#3113=CARTESIAN_POINT('',(11.25,25.,36.4190038418756));
#3114=CARTESIAN_POINT('',(33.75,25.,33.4190038418756));
#3115=CARTESIAN_POINT('Origin',(30.75,25.,33.4190038418756));
#3116=CARTESIAN_POINT('',(33.75,25.,36.4190038418755));
#3117=CARTESIAN_POINT('',(11.25,25.,33.4190038418756));
#3118=CARTESIAN_POINT('',(11.25,25.,36.4190038418756));
#3119=CARTESIAN_POINT('Origin',(14.25,25.,33.4190038418756));
#3120=CARTESIAN_POINT('Origin',(11.25,25.,36.4190038418756));
#3121=CARTESIAN_POINT('',(11.25,16.,13.9190038418755));
#3122=CARTESIAN_POINT('',(11.25,16.,33.4190038418756));
#3123=CARTESIAN_POINT('',(11.25,16.,13.9190038418755));
#3124=CARTESIAN_POINT('',(11.25,25.,33.4190038418756));
#3125=CARTESIAN_POINT('',(11.25,3.99999999999999,33.4190038418756));
#3126=CARTESIAN_POINT('',(11.25,25.,33.4190038418756));
#3127=CARTESIAN_POINT('',(11.25,4.,13.9190038418755));
#3128=CARTESIAN_POINT('',(11.25,4.,13.9190038418755));
#3129=CARTESIAN_POINT('',(11.25,-5.,13.9190038418755));
#3130=CARTESIAN_POINT('Origin',(33.75,25.,36.4190038418755));
#3131=CARTESIAN_POINT('',(33.75,16.,33.4190038418755));
#3132=CARTESIAN_POINT('',(33.75,25.,33.4190038418756));
#3133=CARTESIAN_POINT('',(33.75,16.,13.9190038418755));
#3134=CARTESIAN_POINT('',(33.75,16.,13.9190038418755));
#3135=CARTESIAN_POINT('',(33.75,4.,13.9190038418755));
#3136=CARTESIAN_POINT('',(33.7500000000001,-5.,13.9190038418755));
#3137=CARTESIAN_POINT('',(33.75,3.99999999999999,33.4190038418755));
#3138=CARTESIAN_POINT('',(33.75,4.,13.9190038418755));
#3139=CARTESIAN_POINT('',(33.75,25.,33.4190038418756));
#3140=CARTESIAN_POINT('Origin',(-11.25,-5.,36.4190038418755));
#3141=CARTESIAN_POINT('',(30.7500000000001,16.,36.4190038418755));
#3142=CARTESIAN_POINT('',(14.25,16.,36.4190038418755));
#3143=CARTESIAN_POINT('',(-11.25,16.,36.4190038418755));
#3144=CARTESIAN_POINT('',(30.7500000000001,-5.,36.4190038418755));
#3145=CARTESIAN_POINT('',(14.25,-5.,36.4190038418755));
#3146=CARTESIAN_POINT('Origin',(-11.2500000000001,4.,13.9190038418755));
#3147=CARTESIAN_POINT('Origin',(30.75,3.99999999999999,33.4190038418756));
#3148=CARTESIAN_POINT('',(-11.2500000000001,4.,13.9190038418755));
#3149=CARTESIAN_POINT('Origin',(14.25,3.99999999999999,33.4190038418756));
#3150=CARTESIAN_POINT('Origin',(-11.2500000000001,16.,13.9190038418755));
#3151=CARTESIAN_POINT('Origin',(30.75,16.,33.4190038418756));
#3152=CARTESIAN_POINT('Origin',(14.25,16.,33.4190038418756));
#3153=CARTESIAN_POINT('',(-11.2500000000001,16.,13.9190038418755));
#3154=CARTESIAN_POINT('Origin',(-11.2500000000001,-5.,13.9190038418755));
#3155=CARTESIAN_POINT('Origin',(30.75,-5.,33.4190038418756));
#3156=CARTESIAN_POINT('Origin',(30.75,-5.,33.4190038418756));
#3157=CARTESIAN_POINT('Origin',(14.25,-5.,33.4190038418756));
#3158=CARTESIAN_POINT('Origin',(14.25,-5.,33.4190038418756));
#3194=UNCERTAINTY_MEASURE_WITH_UNIT(LENGTH_MEASURE(0.01),#3207,
'DISTANCE_ACCURACY_VALUE',
'Maximum model space distance between geometric entities at asserted c
onnectivities');
#3196=UNCERTAINTY_MEASURE_WITH_UNIT(LENGTH_MEASURE(0.01),#3207,
'DISTANCE_ACCURACY_VALUE',
'Maximum model space distance between geometric entities at asserted c
onnectivities');
#3204=(
GEOMETRIC_REPRESENTATION_CONTEXT(3)
GLOBAL_UNCERTAINTY_ASSIGNED_CONTEXT((#3194))
GLOBAL_UNIT_ASSIGNED_CONTEXT((#3207,#3209,#3210))
REPRESENTATION_CONTEXT('','3D')
);
#3206=(
GEOMETRIC_REPRESENTATION_CONTEXT(3)
GLOBAL_UNCERTAINTY_ASSIGNED_CONTEXT((#3196))
GLOBAL_UNIT_ASSIGNED_CONTEXT((#3207,#3209,#3210))
REPRESENTATION_CONTEXT('','3D')
);
#3207=(
LENGTH_UNIT()
NAMED_UNIT(*)
SI_UNIT(.MILLI.,.METRE.)
);
#3209=(
NAMED_UNIT(*)
PLANE_ANGLE_UNIT()
SI_UNIT($,.RADIAN.)
);
#3210=(
NAMED_UNIT(*)
SI_UNIT($,.STERADIAN.)
SOLID_ANGLE_UNIT()
);
#3218=SHAPE_DEFINITION_REPRESENTATION(#3227,#3245);
#3227=PRODUCT_DEFINITION_SHAPE('',$,#3255);
#3245=SHAPE_REPRESENTATION('',(#2016),#3204);
#3247=PRODUCT_DEFINITION_CONTEXT('part definition',#3276,'design');
#3255=PRODUCT_DEFINITION('Angle Bracket','Angle Bracket',#3264,#3247);
#3264=PRODUCT_DEFINITION_FORMATION('',$,#3285);
#3276=APPLICATION_CONTEXT(
'Core Data for Automotive Mechanical Design Process');
#3277=PRODUCT_CONTEXT('part definition',#3276,'mechanical');
#3285=PRODUCT('Angle Bracket','Angle Bracket',$,(#3277));
#3290=PRESENTATION_STYLE_ASSIGNMENT((#3294));
#3294=SURFACE_STYLE_USAGE(.BOTH.,#3298);
#3298=SURFACE_SIDE_STYLE('',(#3302));
#3302=SURFACE_STYLE_FILL_AREA(#3306);
#3306=FILL_AREA_STYLE('Opaque(227,224,212)',(#3310));
#3310=FILL_AREA_STYLE_COLOUR('Opaque(227,224,212)',#3314);
#3314=COLOUR_RGB('Opaque(227,224,212)',0.890196078431372,0.87843137254902,
0.831372549019608);
ENDSEC;
END-ISO-10303-21;
